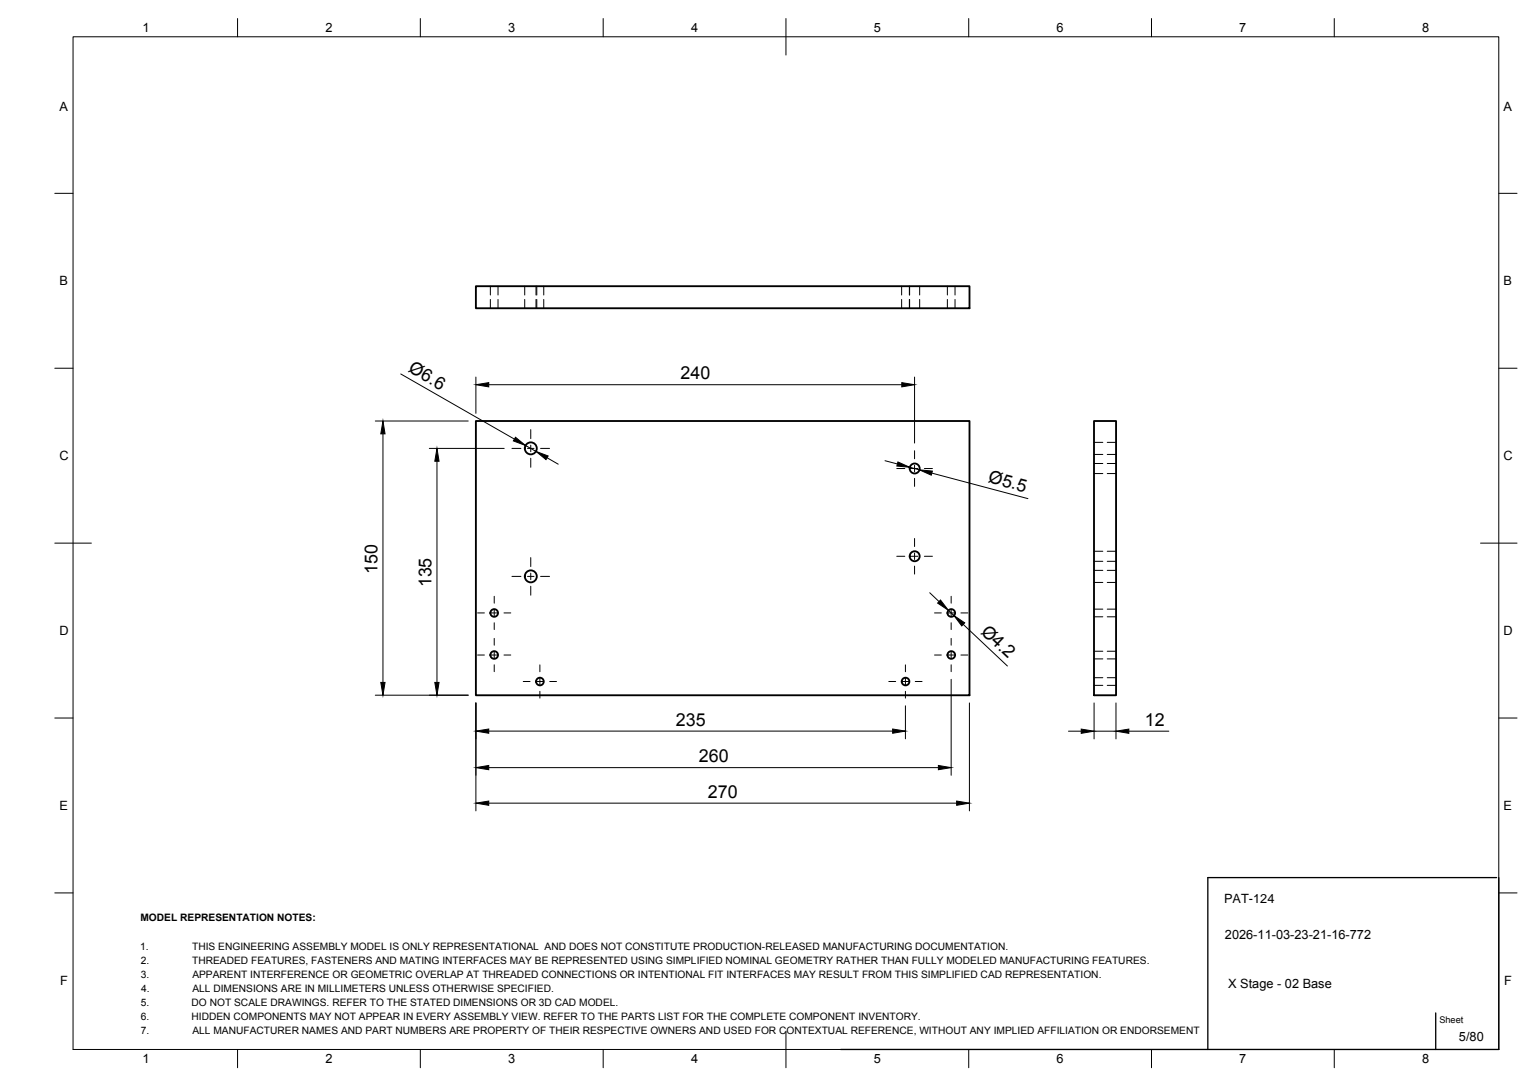
ISO-10303-21;
HEADER;
/* Generated by software containing ST-Developer
 * from STEP Tools, Inc. (www.steptools.com) 
 */

FILE_DESCRIPTION(
/* description */ ('XY cross-slide table'),
/* implementation_level */ '2;1');

FILE_NAME(
/* name */ 'X Stage - 02 Base.step',
/* time_stamp */ '2026-10-28T03:22:46-07:00',
/* author */ (''),
/* organization */ (''),
/* preprocessor_version */ 'ST-DEVELOPER v20.2',
/* originating_system */ 'Autodesk Translation Framework v15.17.0.0',
/* authorisation */ '');

FILE_SCHEMA (('AUTOMOTIVE_DESIGN { 1 0 10303 214 3 1 1 }'));
ENDSEC;

DATA;
#10=MECHANICAL_DESIGN_GEOMETRIC_PRESENTATION_REPRESENTATION('',(#1670),#62984);
#1504=SHAPE_REPRESENTATION_RELATIONSHIP('SRR','None',#63352,#1587);
#1587=ADVANCED_BREP_SHAPE_REPRESENTATION('',(#1783),#62889);
#1670=STYLED_ITEM('',(#63891),#1783);
#1783=MANIFOLD_SOLID_BREP('Body1',#22964);
#1887=FACE_BOUND('',#4198,.T.);
#1888=FACE_BOUND('',#4199,.T.);
#1889=FACE_BOUND('',#4200,.T.);
#1890=FACE_BOUND('',#4201,.T.);
#1891=FACE_BOUND('',#4202,.T.);
#1892=FACE_BOUND('',#4203,.T.);
#1893=FACE_BOUND('',#4204,.T.);
#1894=FACE_BOUND('',#4205,.T.);
#1895=FACE_BOUND('',#4206,.T.);
#1896=FACE_BOUND('',#4207,.T.);
#1897=FACE_BOUND('',#4209,.T.);
#1898=FACE_BOUND('',#4210,.T.);
#1899=FACE_BOUND('',#4211,.T.);
#1900=FACE_BOUND('',#4212,.T.);
#1901=FACE_BOUND('',#4213,.T.);
#1902=FACE_BOUND('',#4214,.T.);
#1903=FACE_BOUND('',#4215,.T.);
#1904=FACE_BOUND('',#4216,.T.);
#1905=FACE_BOUND('',#4217,.T.);
#1906=FACE_BOUND('',#4218,.T.);
#2296=PLANE('',#24034);
#2297=PLANE('',#24035);
#2298=PLANE('',#24036);
#2299=PLANE('',#24037);
#2300=PLANE('',#24038);
#2301=PLANE('',#24039);
#2869=FACE_OUTER_BOUND('',#4183,.T.);
#2870=FACE_OUTER_BOUND('',#4184,.T.);
#2871=FACE_OUTER_BOUND('',#4185,.T.);
#2872=FACE_OUTER_BOUND('',#4186,.T.);
#2873=FACE_OUTER_BOUND('',#4187,.T.);
#2874=FACE_OUTER_BOUND('',#4188,.T.);
#2875=FACE_OUTER_BOUND('',#4189,.T.);
#2876=FACE_OUTER_BOUND('',#4190,.T.);
#2877=FACE_OUTER_BOUND('',#4191,.T.);
#2878=FACE_OUTER_BOUND('',#4192,.T.);
#2879=FACE_OUTER_BOUND('',#4193,.T.);
#2880=FACE_OUTER_BOUND('',#4194,.T.);
#2881=FACE_OUTER_BOUND('',#4195,.T.);
#2882=FACE_OUTER_BOUND('',#4196,.T.);
#2883=FACE_OUTER_BOUND('',#4197,.T.);
#2884=FACE_OUTER_BOUND('',#4208,.T.);
#4183=EDGE_LOOP('',(#14904,#14905,#14906,#14907));
#4184=EDGE_LOOP('',(#14908,#14909,#14910,#14911));
#4185=EDGE_LOOP('',(#14912,#14913,#14914,#14915));
#4186=EDGE_LOOP('',(#14916,#14917,#14918,#14919));
#4187=EDGE_LOOP('',(#14920,#14921,#14922,#14923));
#4188=EDGE_LOOP('',(#14924,#14925,#14926,#14927));
#4189=EDGE_LOOP('',(#14928,#14929,#14930,#14931));
#4190=EDGE_LOOP('',(#14932,#14933,#14934,#14935));
#4191=EDGE_LOOP('',(#14936,#14937,#14938,#14939));
#4192=EDGE_LOOP('',(#14940,#14941,#14942,#14943));
#4193=EDGE_LOOP('',(#14944,#14945,#14946,#14947));
#4194=EDGE_LOOP('',(#14948,#14949,#14950,#14951));
#4195=EDGE_LOOP('',(#14952,#14953,#14954,#14955));
#4196=EDGE_LOOP('',(#14956,#14957,#14958,#14959));
#4197=EDGE_LOOP('',(#14960,#14961,#14962,#14963));
#4198=EDGE_LOOP('',(#14964));
#4199=EDGE_LOOP('',(#14965));
#4200=EDGE_LOOP('',(#14966));
#4201=EDGE_LOOP('',(#14967));
#4202=EDGE_LOOP('',(#14968));
#4203=EDGE_LOOP('',(#14969));
#4204=EDGE_LOOP('',(#14970));
#4205=EDGE_LOOP('',(#14971));
#4206=EDGE_LOOP('',(#14972));
#4207=EDGE_LOOP('',(#14973));
#4208=EDGE_LOOP('',(#14974,#14975,#14976,#14977));
#4209=EDGE_LOOP('',(#14978));
#4210=EDGE_LOOP('',(#14979));
#4211=EDGE_LOOP('',(#14980));
#4212=EDGE_LOOP('',(#14981));
#4213=EDGE_LOOP('',(#14982));
#4214=EDGE_LOOP('',(#14983));
#4215=EDGE_LOOP('',(#14984));
#4216=EDGE_LOOP('',(#14985));
#4217=EDGE_LOOP('',(#14986));
#4218=EDGE_LOOP('',(#14987));
#5906=LINE('',#32878,#7393);
#5907=LINE('',#32884,#7394);
#5908=LINE('',#32890,#7395);
#5909=LINE('',#32896,#7396);
#5910=LINE('',#32902,#7397);
#5911=LINE('',#32908,#7398);
#5912=LINE('',#32914,#7399);
#5913=LINE('',#32920,#7400);
#5914=LINE('',#32926,#7401);
#5915=LINE('',#32932,#7402);
#5916=LINE('',#32937,#7403);
#5917=LINE('',#32939,#7404);
#5918=LINE('',#32941,#7405);
#5919=LINE('',#32942,#7406);
#5920=LINE('',#32945,#7407);
#5921=LINE('',#32947,#7408);
#5922=LINE('',#32948,#7409);
#5923=LINE('',#32951,#7410);
#5924=LINE('',#32953,#7411);
#5925=LINE('',#32954,#7412);
#5926=LINE('',#32956,#7413);
#5927=LINE('',#32957,#7414);
#7393=VECTOR('',#26473,0.210000000000001);
#7394=VECTOR('',#26480,0.21);
#7395=VECTOR('',#26487,0.329999999999998);
#7396=VECTOR('',#26494,0.329999999999998);
#7397=VECTOR('',#26501,0.275);
#7398=VECTOR('',#26508,0.275);
#7399=VECTOR('',#26515,0.210000000000001);
#7400=VECTOR('',#26522,0.21);
#7401=VECTOR('',#26529,0.21);
#7402=VECTOR('',#26536,0.210000000000001);
#7403=VECTOR('',#26541,1.);
#7404=VECTOR('',#26542,1.);
#7405=VECTOR('',#26543,1.);
#7406=VECTOR('',#26544,1.);
#7407=VECTOR('',#26547,1.);
#7408=VECTOR('',#26548,1.);
#7409=VECTOR('',#26549,1.);
#7410=VECTOR('',#26552,1.);
#7411=VECTOR('',#26553,1.);
#7412=VECTOR('',#26554,1.);
#7413=VECTOR('',#26557,1.);
#7414=VECTOR('',#26558,1.);
#8880=CIRCLE('',#24005,0.210000000000001);
#8881=CIRCLE('',#24006,0.210000000000001);
#8882=CIRCLE('',#24008,0.21);
#8883=CIRCLE('',#24009,0.21);
#8884=CIRCLE('',#24011,0.329999999999998);
#8885=CIRCLE('',#24012,0.329999999999998);
#8886=CIRCLE('',#24014,0.329999999999998);
#8887=CIRCLE('',#24015,0.329999999999998);
#8888=CIRCLE('',#24017,0.275);
#8889=CIRCLE('',#24018,0.275);
#8890=CIRCLE('',#24020,0.275);
#8891=CIRCLE('',#24021,0.275);
#8892=CIRCLE('',#24023,0.210000000000001);
#8893=CIRCLE('',#24024,0.210000000000001);
#8894=CIRCLE('',#24026,0.21);
#8895=CIRCLE('',#24027,0.21);
#8896=CIRCLE('',#24029,0.21);
#8897=CIRCLE('',#24030,0.21);
#8898=CIRCLE('',#24032,0.210000000000001);
#8899=CIRCLE('',#24033,0.210000000000001);
#9773=VERTEX_POINT('',#32875);
#9774=VERTEX_POINT('',#32877);
#9775=VERTEX_POINT('',#32881);
#9776=VERTEX_POINT('',#32883);
#9777=VERTEX_POINT('',#32887);
#9778=VERTEX_POINT('',#32889);
#9779=VERTEX_POINT('',#32893);
#9780=VERTEX_POINT('',#32895);
#9781=VERTEX_POINT('',#32899);
#9782=VERTEX_POINT('',#32901);
#9783=VERTEX_POINT('',#32905);
#9784=VERTEX_POINT('',#32907);
#9785=VERTEX_POINT('',#32911);
#9786=VERTEX_POINT('',#32913);
#9787=VERTEX_POINT('',#32917);
#9788=VERTEX_POINT('',#32919);
#9789=VERTEX_POINT('',#32923);
#9790=VERTEX_POINT('',#32925);
#9791=VERTEX_POINT('',#32929);
#9792=VERTEX_POINT('',#32931);
#9793=VERTEX_POINT('',#32935);
#9794=VERTEX_POINT('',#32936);
#9795=VERTEX_POINT('',#32938);
#9796=VERTEX_POINT('',#32940);
#9797=VERTEX_POINT('',#32944);
#9798=VERTEX_POINT('',#32946);
#9799=VERTEX_POINT('',#32950);
#9800=VERTEX_POINT('',#32952);
#11836=EDGE_CURVE('',#9773,#9773,#8880,.T.);
#11837=EDGE_CURVE('',#9773,#9774,#5906,.T.);
#11838=EDGE_CURVE('',#9774,#9774,#8881,.T.);
#11839=EDGE_CURVE('',#9775,#9775,#8882,.T.);
#11840=EDGE_CURVE('',#9775,#9776,#5907,.T.);
#11841=EDGE_CURVE('',#9776,#9776,#8883,.T.);
#11842=EDGE_CURVE('',#9777,#9777,#8884,.T.);
#11843=EDGE_CURVE('',#9777,#9778,#5908,.T.);
#11844=EDGE_CURVE('',#9778,#9778,#8885,.T.);
#11845=EDGE_CURVE('',#9779,#9779,#8886,.T.);
#11846=EDGE_CURVE('',#9779,#9780,#5909,.T.);
#11847=EDGE_CURVE('',#9780,#9780,#8887,.T.);
#11848=EDGE_CURVE('',#9781,#9781,#8888,.T.);
#11849=EDGE_CURVE('',#9781,#9782,#5910,.T.);
#11850=EDGE_CURVE('',#9782,#9782,#8889,.T.);
#11851=EDGE_CURVE('',#9783,#9783,#8890,.T.);
#11852=EDGE_CURVE('',#9783,#9784,#5911,.T.);
#11853=EDGE_CURVE('',#9784,#9784,#8891,.T.);
#11854=EDGE_CURVE('',#9785,#9785,#8892,.T.);
#11855=EDGE_CURVE('',#9785,#9786,#5912,.T.);
#11856=EDGE_CURVE('',#9786,#9786,#8893,.T.);
#11857=EDGE_CURVE('',#9787,#9787,#8894,.T.);
#11858=EDGE_CURVE('',#9787,#9788,#5913,.T.);
#11859=EDGE_CURVE('',#9788,#9788,#8895,.T.);
#11860=EDGE_CURVE('',#9789,#9789,#8896,.T.);
#11861=EDGE_CURVE('',#9789,#9790,#5914,.T.);
#11862=EDGE_CURVE('',#9790,#9790,#8897,.T.);
#11863=EDGE_CURVE('',#9791,#9791,#8898,.T.);
#11864=EDGE_CURVE('',#9791,#9792,#5915,.T.);
#11865=EDGE_CURVE('',#9792,#9792,#8899,.T.);
#11866=EDGE_CURVE('',#9793,#9794,#5916,.T.);
#11867=EDGE_CURVE('',#9794,#9795,#5917,.T.);
#11868=EDGE_CURVE('',#9796,#9795,#5918,.T.);
#11869=EDGE_CURVE('',#9793,#9796,#5919,.T.);
#11870=EDGE_CURVE('',#9797,#9793,#5920,.T.);
#11871=EDGE_CURVE('',#9798,#9796,#5921,.T.);
#11872=EDGE_CURVE('',#9797,#9798,#5922,.T.);
#11873=EDGE_CURVE('',#9799,#9797,#5923,.T.);
#11874=EDGE_CURVE('',#9800,#9798,#5924,.T.);
#11875=EDGE_CURVE('',#9799,#9800,#5925,.T.);
#11876=EDGE_CURVE('',#9794,#9799,#5926,.T.);
#11877=EDGE_CURVE('',#9795,#9800,#5927,.T.);
#14904=ORIENTED_EDGE('',*,*,#11836,.F.);
#14905=ORIENTED_EDGE('',*,*,#11837,.T.);
#14906=ORIENTED_EDGE('',*,*,#11838,.F.);
#14907=ORIENTED_EDGE('',*,*,#11837,.F.);
#14908=ORIENTED_EDGE('',*,*,#11839,.F.);
#14909=ORIENTED_EDGE('',*,*,#11840,.T.);
#14910=ORIENTED_EDGE('',*,*,#11841,.F.);
#14911=ORIENTED_EDGE('',*,*,#11840,.F.);
#14912=ORIENTED_EDGE('',*,*,#11842,.F.);
#14913=ORIENTED_EDGE('',*,*,#11843,.T.);
#14914=ORIENTED_EDGE('',*,*,#11844,.F.);
#14915=ORIENTED_EDGE('',*,*,#11843,.F.);
#14916=ORIENTED_EDGE('',*,*,#11845,.F.);
#14917=ORIENTED_EDGE('',*,*,#11846,.T.);
#14918=ORIENTED_EDGE('',*,*,#11847,.F.);
#14919=ORIENTED_EDGE('',*,*,#11846,.F.);
#14920=ORIENTED_EDGE('',*,*,#11848,.F.);
#14921=ORIENTED_EDGE('',*,*,#11849,.T.);
#14922=ORIENTED_EDGE('',*,*,#11850,.F.);
#14923=ORIENTED_EDGE('',*,*,#11849,.F.);
#14924=ORIENTED_EDGE('',*,*,#11851,.F.);
#14925=ORIENTED_EDGE('',*,*,#11852,.T.);
#14926=ORIENTED_EDGE('',*,*,#11853,.F.);
#14927=ORIENTED_EDGE('',*,*,#11852,.F.);
#14928=ORIENTED_EDGE('',*,*,#11854,.F.);
#14929=ORIENTED_EDGE('',*,*,#11855,.T.);
#14930=ORIENTED_EDGE('',*,*,#11856,.F.);
#14931=ORIENTED_EDGE('',*,*,#11855,.F.);
#14932=ORIENTED_EDGE('',*,*,#11857,.F.);
#14933=ORIENTED_EDGE('',*,*,#11858,.T.);
#14934=ORIENTED_EDGE('',*,*,#11859,.F.);
#14935=ORIENTED_EDGE('',*,*,#11858,.F.);
#14936=ORIENTED_EDGE('',*,*,#11860,.F.);
#14937=ORIENTED_EDGE('',*,*,#11861,.T.);
#14938=ORIENTED_EDGE('',*,*,#11862,.F.);
#14939=ORIENTED_EDGE('',*,*,#11861,.F.);
#14940=ORIENTED_EDGE('',*,*,#11863,.F.);
#14941=ORIENTED_EDGE('',*,*,#11864,.T.);
#14942=ORIENTED_EDGE('',*,*,#11865,.F.);
#14943=ORIENTED_EDGE('',*,*,#11864,.F.);
#14944=ORIENTED_EDGE('',*,*,#11866,.T.);
#14945=ORIENTED_EDGE('',*,*,#11867,.T.);
#14946=ORIENTED_EDGE('',*,*,#11868,.F.);
#14947=ORIENTED_EDGE('',*,*,#11869,.F.);
#14948=ORIENTED_EDGE('',*,*,#11870,.T.);
#14949=ORIENTED_EDGE('',*,*,#11869,.T.);
#14950=ORIENTED_EDGE('',*,*,#11871,.F.);
#14951=ORIENTED_EDGE('',*,*,#11872,.F.);
#14952=ORIENTED_EDGE('',*,*,#11873,.T.);
#14953=ORIENTED_EDGE('',*,*,#11872,.T.);
#14954=ORIENTED_EDGE('',*,*,#11874,.F.);
#14955=ORIENTED_EDGE('',*,*,#11875,.F.);
#14956=ORIENTED_EDGE('',*,*,#11876,.T.);
#14957=ORIENTED_EDGE('',*,*,#11875,.T.);
#14958=ORIENTED_EDGE('',*,*,#11877,.F.);
#14959=ORIENTED_EDGE('',*,*,#11867,.F.);
#14960=ORIENTED_EDGE('',*,*,#11877,.T.);
#14961=ORIENTED_EDGE('',*,*,#11874,.T.);
#14962=ORIENTED_EDGE('',*,*,#11871,.T.);
#14963=ORIENTED_EDGE('',*,*,#11868,.T.);
#14964=ORIENTED_EDGE('',*,*,#11841,.T.);
#14965=ORIENTED_EDGE('',*,*,#11865,.T.);
#14966=ORIENTED_EDGE('',*,*,#11862,.T.);
#14967=ORIENTED_EDGE('',*,*,#11859,.T.);
#14968=ORIENTED_EDGE('',*,*,#11856,.T.);
#14969=ORIENTED_EDGE('',*,*,#11853,.T.);
#14970=ORIENTED_EDGE('',*,*,#11850,.T.);
#14971=ORIENTED_EDGE('',*,*,#11847,.T.);
#14972=ORIENTED_EDGE('',*,*,#11844,.T.);
#14973=ORIENTED_EDGE('',*,*,#11838,.T.);
#14974=ORIENTED_EDGE('',*,*,#11876,.F.);
#14975=ORIENTED_EDGE('',*,*,#11866,.F.);
#14976=ORIENTED_EDGE('',*,*,#11870,.F.);
#14977=ORIENTED_EDGE('',*,*,#11873,.F.);
#14978=ORIENTED_EDGE('',*,*,#11839,.T.);
#14979=ORIENTED_EDGE('',*,*,#11863,.T.);
#14980=ORIENTED_EDGE('',*,*,#11860,.T.);
#14981=ORIENTED_EDGE('',*,*,#11857,.T.);
#14982=ORIENTED_EDGE('',*,*,#11854,.T.);
#14983=ORIENTED_EDGE('',*,*,#11851,.T.);
#14984=ORIENTED_EDGE('',*,*,#11848,.T.);
#14985=ORIENTED_EDGE('',*,*,#11845,.T.);
#14986=ORIENTED_EDGE('',*,*,#11842,.T.);
#14987=ORIENTED_EDGE('',*,*,#11836,.T.);
#21040=CYLINDRICAL_SURFACE('',#24004,0.210000000000001);
#21041=CYLINDRICAL_SURFACE('',#24007,0.21);
#21042=CYLINDRICAL_SURFACE('',#24010,0.329999999999998);
#21043=CYLINDRICAL_SURFACE('',#24013,0.329999999999998);
#21044=CYLINDRICAL_SURFACE('',#24016,0.275);
#21045=CYLINDRICAL_SURFACE('',#24019,0.275);
#21046=CYLINDRICAL_SURFACE('',#24022,0.210000000000001);
#21047=CYLINDRICAL_SURFACE('',#24025,0.21);
#21048=CYLINDRICAL_SURFACE('',#24028,0.21);
#21049=CYLINDRICAL_SURFACE('',#24031,0.210000000000001);
#21650=ADVANCED_FACE('',(#2869),#21040,.F.);
#21651=ADVANCED_FACE('',(#2870),#21041,.F.);
#21652=ADVANCED_FACE('',(#2871),#21042,.F.);
#21653=ADVANCED_FACE('',(#2872),#21043,.F.);
#21654=ADVANCED_FACE('',(#2873),#21044,.F.);
#21655=ADVANCED_FACE('',(#2874),#21045,.F.);
#21656=ADVANCED_FACE('',(#2875),#21046,.F.);
#21657=ADVANCED_FACE('',(#2876),#21047,.F.);
#21658=ADVANCED_FACE('',(#2877),#21048,.F.);
#21659=ADVANCED_FACE('',(#2878),#21049,.F.);
#21660=ADVANCED_FACE('',(#2879),#2296,.T.);
#21661=ADVANCED_FACE('',(#2880),#2297,.T.);
#21662=ADVANCED_FACE('',(#2881),#2298,.T.);
#21663=ADVANCED_FACE('',(#2882),#2299,.T.);
#21664=ADVANCED_FACE('',(#2883,#1887,#1888,#1889,#1890,#1891,#1892,#1893,
#1894,#1895,#1896),#2300,.T.);
#21665=ADVANCED_FACE('',(#2884,#1897,#1898,#1899,#1900,#1901,#1902,#1903,
#1904,#1905,#1906),#2301,.F.);
#22964=CLOSED_SHELL('',(#21650,#21651,#21652,#21653,#21654,#21655,#21656,
#21657,#21658,#21659,#21660,#21661,#21662,#21663,#21664,#21665));
#24003=AXIS2_PLACEMENT_3D('',#32873,#26467,#26468);
#24004=AXIS2_PLACEMENT_3D('',#32874,#26469,#26470);
#24005=AXIS2_PLACEMENT_3D('',#32876,#26471,#26472);
#24006=AXIS2_PLACEMENT_3D('',#32879,#26474,#26475);
#24007=AXIS2_PLACEMENT_3D('',#32880,#26476,#26477);
#24008=AXIS2_PLACEMENT_3D('',#32882,#26478,#26479);
#24009=AXIS2_PLACEMENT_3D('',#32885,#26481,#26482);
#24010=AXIS2_PLACEMENT_3D('',#32886,#26483,#26484);
#24011=AXIS2_PLACEMENT_3D('',#32888,#26485,#26486);
#24012=AXIS2_PLACEMENT_3D('',#32891,#26488,#26489);
#24013=AXIS2_PLACEMENT_3D('',#32892,#26490,#26491);
#24014=AXIS2_PLACEMENT_3D('',#32894,#26492,#26493);
#24015=AXIS2_PLACEMENT_3D('',#32897,#26495,#26496);
#24016=AXIS2_PLACEMENT_3D('',#32898,#26497,#26498);
#24017=AXIS2_PLACEMENT_3D('',#32900,#26499,#26500);
#24018=AXIS2_PLACEMENT_3D('',#32903,#26502,#26503);
#24019=AXIS2_PLACEMENT_3D('',#32904,#26504,#26505);
#24020=AXIS2_PLACEMENT_3D('',#32906,#26506,#26507);
#24021=AXIS2_PLACEMENT_3D('',#32909,#26509,#26510);
#24022=AXIS2_PLACEMENT_3D('',#32910,#26511,#26512);
#24023=AXIS2_PLACEMENT_3D('',#32912,#26513,#26514);
#24024=AXIS2_PLACEMENT_3D('',#32915,#26516,#26517);
#24025=AXIS2_PLACEMENT_3D('',#32916,#26518,#26519);
#24026=AXIS2_PLACEMENT_3D('',#32918,#26520,#26521);
#24027=AXIS2_PLACEMENT_3D('',#32921,#26523,#26524);
#24028=AXIS2_PLACEMENT_3D('',#32922,#26525,#26526);
#24029=AXIS2_PLACEMENT_3D('',#32924,#26527,#26528);
#24030=AXIS2_PLACEMENT_3D('',#32927,#26530,#26531);
#24031=AXIS2_PLACEMENT_3D('',#32928,#26532,#26533);
#24032=AXIS2_PLACEMENT_3D('',#32930,#26534,#26535);
#24033=AXIS2_PLACEMENT_3D('',#32933,#26537,#26538);
#24034=AXIS2_PLACEMENT_3D('',#32934,#26539,#26540);
#24035=AXIS2_PLACEMENT_3D('',#32943,#26545,#26546);
#24036=AXIS2_PLACEMENT_3D('',#32949,#26550,#26551);
#24037=AXIS2_PLACEMENT_3D('',#32955,#26555,#26556);
#24038=AXIS2_PLACEMENT_3D('',#32958,#26559,#26560);
#24039=AXIS2_PLACEMENT_3D('',#32959,#26561,#26562);
#26467=DIRECTION('axis',(0.,0.,1.));
#26468=DIRECTION('refdir',(1.,0.,0.));
#26469=DIRECTION('center_axis',(0.,0.,1.));
#26470=DIRECTION('ref_axis',(1.,0.,0.));
#26471=DIRECTION('center_axis',(0.,0.,1.));
#26472=DIRECTION('ref_axis',(1.,0.,0.));
#26473=DIRECTION('',(0.,0.,1.));
#26474=DIRECTION('center_axis',(0.,0.,-1.));
#26475=DIRECTION('ref_axis',(1.,0.,0.));
#26476=DIRECTION('center_axis',(0.,0.,1.));
#26477=DIRECTION('ref_axis',(1.,0.,0.));
#26478=DIRECTION('center_axis',(0.,0.,1.));
#26479=DIRECTION('ref_axis',(1.,0.,0.));
#26480=DIRECTION('',(0.,0.,1.));
#26481=DIRECTION('center_axis',(0.,0.,-1.));
#26482=DIRECTION('ref_axis',(1.,0.,0.));
#26483=DIRECTION('center_axis',(0.,0.,1.));
#26484=DIRECTION('ref_axis',(1.,0.,0.));
#26485=DIRECTION('center_axis',(0.,0.,1.));
#26486=DIRECTION('ref_axis',(1.,0.,0.));
#26487=DIRECTION('',(0.,0.,1.));
#26488=DIRECTION('center_axis',(0.,0.,-1.));
#26489=DIRECTION('ref_axis',(1.,0.,0.));
#26490=DIRECTION('center_axis',(0.,0.,1.));
#26491=DIRECTION('ref_axis',(1.,0.,0.));
#26492=DIRECTION('center_axis',(0.,0.,1.));
#26493=DIRECTION('ref_axis',(1.,0.,0.));
#26494=DIRECTION('',(0.,0.,1.));
#26495=DIRECTION('center_axis',(0.,0.,-1.));
#26496=DIRECTION('ref_axis',(1.,0.,0.));
#26497=DIRECTION('center_axis',(0.,0.,1.));
#26498=DIRECTION('ref_axis',(1.,0.,0.));
#26499=DIRECTION('center_axis',(0.,0.,1.));
#26500=DIRECTION('ref_axis',(1.,0.,0.));
#26501=DIRECTION('',(0.,0.,1.));
#26502=DIRECTION('center_axis',(0.,0.,-1.));
#26503=DIRECTION('ref_axis',(1.,0.,0.));
#26504=DIRECTION('center_axis',(0.,0.,1.));
#26505=DIRECTION('ref_axis',(1.,0.,0.));
#26506=DIRECTION('center_axis',(0.,0.,1.));
#26507=DIRECTION('ref_axis',(1.,0.,0.));
#26508=DIRECTION('',(0.,0.,1.));
#26509=DIRECTION('center_axis',(0.,0.,-1.));
#26510=DIRECTION('ref_axis',(1.,0.,0.));
#26511=DIRECTION('center_axis',(0.,0.,1.));
#26512=DIRECTION('ref_axis',(1.,0.,0.));
#26513=DIRECTION('center_axis',(0.,0.,1.));
#26514=DIRECTION('ref_axis',(1.,0.,0.));
#26515=DIRECTION('',(0.,0.,1.));
#26516=DIRECTION('center_axis',(0.,0.,-1.));
#26517=DIRECTION('ref_axis',(1.,0.,0.));
#26518=DIRECTION('center_axis',(0.,0.,1.));
#26519=DIRECTION('ref_axis',(1.,0.,0.));
#26520=DIRECTION('center_axis',(0.,0.,1.));
#26521=DIRECTION('ref_axis',(1.,0.,0.));
#26522=DIRECTION('',(0.,0.,1.));
#26523=DIRECTION('center_axis',(0.,0.,-1.));
#26524=DIRECTION('ref_axis',(1.,0.,0.));
#26525=DIRECTION('center_axis',(0.,0.,1.));
#26526=DIRECTION('ref_axis',(1.,0.,0.));
#26527=DIRECTION('center_axis',(0.,0.,1.));
#26528=DIRECTION('ref_axis',(1.,0.,0.));
#26529=DIRECTION('',(0.,0.,1.));
#26530=DIRECTION('center_axis',(0.,0.,-1.));
#26531=DIRECTION('ref_axis',(1.,0.,0.));
#26532=DIRECTION('center_axis',(0.,0.,1.));
#26533=DIRECTION('ref_axis',(1.,0.,0.));
#26534=DIRECTION('center_axis',(0.,0.,1.));
#26535=DIRECTION('ref_axis',(1.,0.,0.));
#26536=DIRECTION('',(0.,0.,1.));
#26537=DIRECTION('center_axis',(0.,0.,-1.));
#26538=DIRECTION('ref_axis',(1.,0.,0.));
#26539=DIRECTION('center_axis',(0.,1.,0.));
#26540=DIRECTION('ref_axis',(-1.,0.,0.));
#26541=DIRECTION('',(-1.,0.,0.));
#26542=DIRECTION('',(0.,0.,1.));
#26543=DIRECTION('',(-1.,0.,0.));
#26544=DIRECTION('',(0.,0.,1.));
#26545=DIRECTION('center_axis',(1.,0.,0.));
#26546=DIRECTION('ref_axis',(0.,1.,0.));
#26547=DIRECTION('',(0.,1.,0.));
#26548=DIRECTION('',(0.,1.,0.));
#26549=DIRECTION('',(0.,0.,1.));
#26550=DIRECTION('center_axis',(0.,-1.,0.));
#26551=DIRECTION('ref_axis',(1.,0.,0.));
#26552=DIRECTION('',(1.,0.,0.));
#26553=DIRECTION('',(1.,0.,0.));
#26554=DIRECTION('',(0.,0.,1.));
#26555=DIRECTION('center_axis',(-1.,0.,0.));
#26556=DIRECTION('ref_axis',(0.,-1.,0.));
#26557=DIRECTION('',(0.,-1.,0.));
#26558=DIRECTION('',(0.,-1.,0.));
#26559=DIRECTION('center_axis',(0.,0.,1.));
#26560=DIRECTION('ref_axis',(1.,0.,0.));
#26561=DIRECTION('center_axis',(0.,0.,1.));
#26562=DIRECTION('ref_axis',(1.,0.,0.));
#32873=CARTESIAN_POINT('',(0.,0.,0.));
#32874=CARTESIAN_POINT('Origin',(23.5,-9.25,-0.1));
#32875=CARTESIAN_POINT('',(23.29,-9.25,0.));
#32876=CARTESIAN_POINT('Origin',(23.5,-9.25,0.));
#32877=CARTESIAN_POINT('',(23.29,-9.25,1.2));
#32878=CARTESIAN_POINT('',(23.29,-9.25,-0.1));
#32879=CARTESIAN_POINT('Origin',(23.5,-9.25,1.2));
#32880=CARTESIAN_POINT('Origin',(3.5,-9.25,-0.1));
#32881=CARTESIAN_POINT('',(3.29,-9.25,0.));
#32882=CARTESIAN_POINT('Origin',(3.5,-9.25,0.));
#32883=CARTESIAN_POINT('',(3.29,-9.25,1.2));
#32884=CARTESIAN_POINT('',(3.29,-9.25,-0.1));
#32885=CARTESIAN_POINT('Origin',(3.5,-9.25,1.2));
#32886=CARTESIAN_POINT('Origin',(24.,-3.5,-0.1));
#32887=CARTESIAN_POINT('',(23.67,-3.5,0.));
#32888=CARTESIAN_POINT('Origin',(24.,-3.5,0.));
#32889=CARTESIAN_POINT('',(23.67,-3.5,1.2));
#32890=CARTESIAN_POINT('',(23.67,-3.5,-0.1));
#32891=CARTESIAN_POINT('Origin',(24.,-3.5,1.2));
#32892=CARTESIAN_POINT('Origin',(24.,3.5,-0.1));
#32893=CARTESIAN_POINT('',(23.67,3.5,0.));
#32894=CARTESIAN_POINT('Origin',(24.,3.5,0.));
#32895=CARTESIAN_POINT('',(23.67,3.5,1.2));
#32896=CARTESIAN_POINT('',(23.67,3.5,-0.1));
#32897=CARTESIAN_POINT('Origin',(24.,3.5,1.2));
#32898=CARTESIAN_POINT('Origin',(3.,-2.4,-0.1));
#32899=CARTESIAN_POINT('',(2.725,-2.4,0.));
#32900=CARTESIAN_POINT('Origin',(3.,-2.4,0.));
#32901=CARTESIAN_POINT('',(2.725,-2.4,1.2));
#32902=CARTESIAN_POINT('',(2.725,-2.4,-0.1));
#32903=CARTESIAN_POINT('Origin',(3.,-2.4,1.2));
#32904=CARTESIAN_POINT('Origin',(3.,2.4,-0.1));
#32905=CARTESIAN_POINT('',(2.725,2.4,0.));
#32906=CARTESIAN_POINT('Origin',(3.,2.4,0.));
#32907=CARTESIAN_POINT('',(2.725,2.4,1.2));
#32908=CARTESIAN_POINT('',(2.725,2.4,-0.1));
#32909=CARTESIAN_POINT('Origin',(3.,2.4,1.2));
#32910=CARTESIAN_POINT('Origin',(26.,-7.8,-0.1));
#32911=CARTESIAN_POINT('',(25.79,-7.8,0.));
#32912=CARTESIAN_POINT('Origin',(26.,-7.8,0.));
#32913=CARTESIAN_POINT('',(25.79,-7.8,1.2));
#32914=CARTESIAN_POINT('',(25.79,-7.8,-0.1));
#32915=CARTESIAN_POINT('Origin',(26.,-7.8,1.2));
#32916=CARTESIAN_POINT('Origin',(1.,-5.5,-0.1));
#32917=CARTESIAN_POINT('',(0.79,-5.5,0.));
#32918=CARTESIAN_POINT('Origin',(1.,-5.5,0.));
#32919=CARTESIAN_POINT('',(0.79,-5.5,1.2));
#32920=CARTESIAN_POINT('',(0.79,-5.5,-0.1));
#32921=CARTESIAN_POINT('Origin',(1.,-5.5,1.2));
#32922=CARTESIAN_POINT('Origin',(1.,-7.8,-0.1));
#32923=CARTESIAN_POINT('',(0.79,-7.8,0.));
#32924=CARTESIAN_POINT('Origin',(1.,-7.8,0.));
#32925=CARTESIAN_POINT('',(0.79,-7.8,1.2));
#32926=CARTESIAN_POINT('',(0.79,-7.8,-0.1));
#32927=CARTESIAN_POINT('Origin',(1.,-7.8,1.2));
#32928=CARTESIAN_POINT('Origin',(26.,-5.5,-0.1));
#32929=CARTESIAN_POINT('',(25.79,-5.5,0.));
#32930=CARTESIAN_POINT('Origin',(26.,-5.5,0.));
#32931=CARTESIAN_POINT('',(25.79,-5.5,1.2));
#32932=CARTESIAN_POINT('',(25.79,-5.5,-0.1));
#32933=CARTESIAN_POINT('Origin',(26.,-5.5,1.2));
#32934=CARTESIAN_POINT('Origin',(27.,5.,0.));
#32935=CARTESIAN_POINT('',(27.,5.,0.));
#32936=CARTESIAN_POINT('',(0.,5.,0.));
#32937=CARTESIAN_POINT('',(27.,5.,0.));
#32938=CARTESIAN_POINT('',(0.,5.,1.2));
#32939=CARTESIAN_POINT('',(0.,5.,0.));
#32940=CARTESIAN_POINT('',(27.,5.,1.2));
#32941=CARTESIAN_POINT('',(27.,5.,1.2));
#32942=CARTESIAN_POINT('',(27.,5.,0.));
#32943=CARTESIAN_POINT('Origin',(27.,-10.,0.));
#32944=CARTESIAN_POINT('',(27.,-10.,0.));
#32945=CARTESIAN_POINT('',(27.,-10.,0.));
#32946=CARTESIAN_POINT('',(27.,-10.,1.2));
#32947=CARTESIAN_POINT('',(27.,-10.,1.2));
#32948=CARTESIAN_POINT('',(27.,-10.,0.));
#32949=CARTESIAN_POINT('Origin',(0.,-10.,0.));
#32950=CARTESIAN_POINT('',(0.,-10.,0.));
#32951=CARTESIAN_POINT('',(0.,-10.,0.));
#32952=CARTESIAN_POINT('',(0.,-10.,1.2));
#32953=CARTESIAN_POINT('',(0.,-10.,1.2));
#32954=CARTESIAN_POINT('',(0.,-10.,0.));
#32955=CARTESIAN_POINT('Origin',(0.,5.,0.));
#32956=CARTESIAN_POINT('',(0.,5.,0.));
#32957=CARTESIAN_POINT('',(0.,5.,1.2));
#32958=CARTESIAN_POINT('Origin',(13.5,-2.5,1.2));
#32959=CARTESIAN_POINT('Origin',(13.5,-2.5,0.));
#62790=UNCERTAINTY_MEASURE_WITH_UNIT(LENGTH_MEASURE(0.001),#62985,
'DISTANCE_ACCURACY_VALUE',
'Maximum model space distance between geometric entities at asserted c
onnectivities');
#62885=UNCERTAINTY_MEASURE_WITH_UNIT(LENGTH_MEASURE(0.001),#62985,
'DISTANCE_ACCURACY_VALUE',
'Maximum model space distance between geometric entities at asserted c
onnectivities');
#62889=(
GEOMETRIC_REPRESENTATION_CONTEXT(3)
GLOBAL_UNCERTAINTY_ASSIGNED_CONTEXT((#62790))
GLOBAL_UNIT_ASSIGNED_CONTEXT((#62985,#62987,#62988))
REPRESENTATION_CONTEXT('','3D')
);
#62984=(
GEOMETRIC_REPRESENTATION_CONTEXT(3)
GLOBAL_UNCERTAINTY_ASSIGNED_CONTEXT((#62885))
GLOBAL_UNIT_ASSIGNED_CONTEXT((#62985,#62987,#62988))
REPRESENTATION_CONTEXT('','3D')
);
#62985=(
LENGTH_UNIT()
NAMED_UNIT(*)
SI_UNIT(.CENTI.,.METRE.)
);
#62987=(
NAMED_UNIT(*)
PLANE_ANGLE_UNIT()
SI_UNIT($,.RADIAN.)
);
#62988=(
NAMED_UNIT(*)
SI_UNIT($,.STERADIAN.)
SOLID_ANGLE_UNIT()
);
#62992=SHAPE_DEFINITION_REPRESENTATION(#63090,#63352);
#63090=PRODUCT_DEFINITION_SHAPE('',$,#63451);
#63352=SHAPE_REPRESENTATION('',(#24003),#62889);
#63447=PRODUCT_DEFINITION_CONTEXT('part definition',#63743,'design');
#63451=PRODUCT_DEFINITION('X Stage - 02 Base','X Stage - 02 Base',#63549,
#63447);
#63549=PRODUCT_DEFINITION_FORMATION('',$,#63748);
#63743=APPLICATION_CONTEXT(
'Core Data for Automotive Mechanical Design Process');
#63744=PRODUCT_CONTEXT('part definition',#63743,'mechanical');
#63748=PRODUCT('X Stage - 02 Base','X Stage - 02 Base',
'X Stage - 02 Base',(#63744));
#63885=COLOUR_RGB('Dark Blue',0.08,0.2,0.34);
#63886=FILL_AREA_STYLE_COLOUR('',#63885);
#63887=FILL_AREA_STYLE('',(#63886));
#63888=SURFACE_STYLE_FILL_AREA(#63887);
#63889=SURFACE_SIDE_STYLE('',(#63888));
#63890=SURFACE_STYLE_USAGE(.BOTH.,#63889);
#63891=PRESENTATION_STYLE_ASSIGNMENT((#63890));
ENDSEC;
END-ISO-10303-21;
